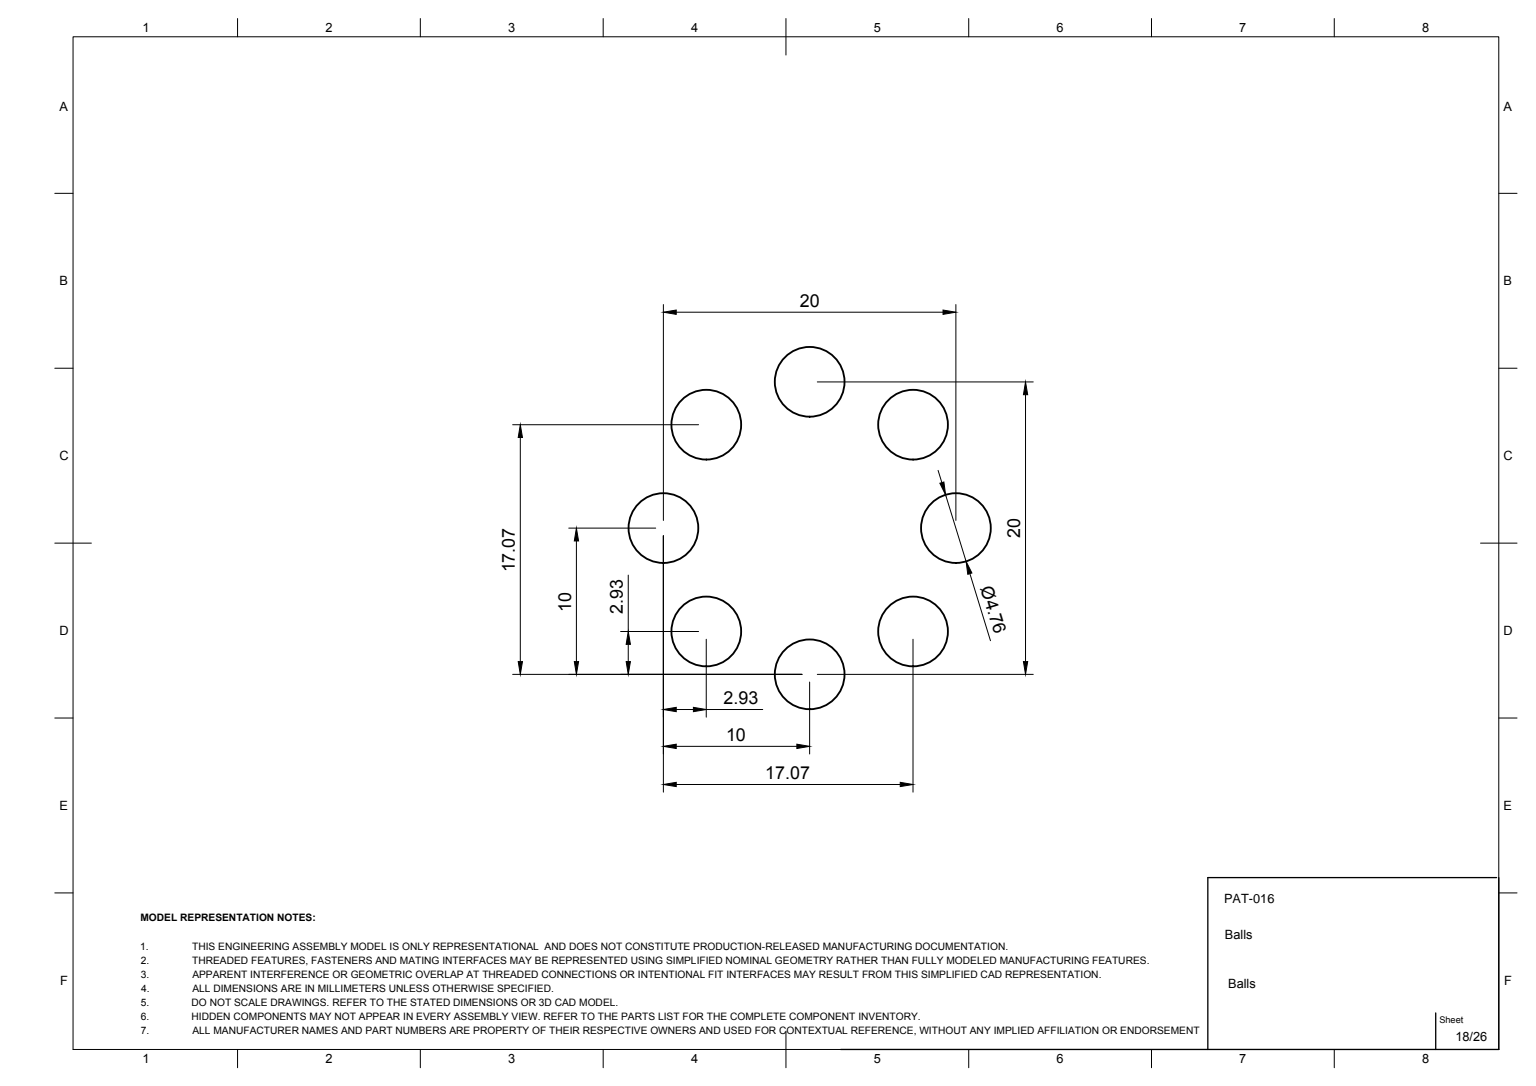
ISO-10303-21;
HEADER;
/* Generated by software containing ST-Developer
 * from STEP Tools, Inc. (www.steptools.com) 
 */

FILE_DESCRIPTION(
/* description */ ('Bracket-mounted idler roller'),
/* implementation_level */ '2;1');

FILE_NAME(
/* name */ 'Balls.step',
/* time_stamp */ '2026-10-28T03:26:42-07:00',
/* author */ (''),
/* organization */ (''),
/* preprocessor_version */ 'ST-DEVELOPER v20.2',
/* originating_system */ 'Autodesk Translation Framework v15.17.0.0',
/* authorisation */ '');

FILE_SCHEMA (('AUTOMOTIVE_DESIGN { 1 0 10303 214 3 1 1 }'));
ENDSEC;

DATA;
#10=MECHANICAL_DESIGN_GEOMETRIC_PRESENTATION_REPRESENTATION('',(#293,#294,#295,#296,#297,#298,#299,#300),#6241);
#205=SPHERICAL_SURFACE('',#3648,0.23815);
#206=SPHERICAL_SURFACE('',#3650,0.23815);
#207=SPHERICAL_SURFACE('',#3652,0.23815);
#208=SPHERICAL_SURFACE('',#3654,0.23815);
#209=SPHERICAL_SURFACE('',#3656,0.23815);
#210=SPHERICAL_SURFACE('',#3658,0.23815);
#211=SPHERICAL_SURFACE('',#3660,0.23815);
#212=SPHERICAL_SURFACE('',#3662,0.23815);
#251=SHAPE_REPRESENTATION_RELATIONSHIP('SRR','None',#6356,#272);
#272=ADVANCED_BREP_SHAPE_REPRESENTATION('',(#321,#322,#323,#324,#325,#326,
#327,#328),#6232);
#293=STYLED_ITEM('',(#6538),#321);
#294=STYLED_ITEM('',(#6538),#322);
#295=STYLED_ITEM('',(#6538),#323);
#296=STYLED_ITEM('',(#6538),#324);
#297=STYLED_ITEM('',(#6538),#325);
#298=STYLED_ITEM('',(#6538),#326);
#299=STYLED_ITEM('',(#6538),#327);
#300=STYLED_ITEM('',(#6538),#328);
#321=MANIFOLD_SOLID_BREP('Body1',#3196);
#322=MANIFOLD_SOLID_BREP('Body2',#3197);
#323=MANIFOLD_SOLID_BREP('Body3',#3198);
#324=MANIFOLD_SOLID_BREP('Body4',#3199);
#325=MANIFOLD_SOLID_BREP('Body5',#3200);
#326=MANIFOLD_SOLID_BREP('Body6',#3201);
#327=MANIFOLD_SOLID_BREP('Body7',#3202);
#328=MANIFOLD_SOLID_BREP('Body8',#3203);
#623=FACE_OUTER_BOUND('',#855,.T.);
#624=FACE_OUTER_BOUND('',#856,.T.);
#625=FACE_OUTER_BOUND('',#857,.T.);
#626=FACE_OUTER_BOUND('',#858,.T.);
#627=FACE_OUTER_BOUND('',#859,.T.);
#628=FACE_OUTER_BOUND('',#860,.T.);
#629=FACE_OUTER_BOUND('',#861,.T.);
#630=FACE_OUTER_BOUND('',#862,.T.);
#855=EDGE_LOOP('',(#2584,#2585));
#856=EDGE_LOOP('',(#2586,#2587));
#857=EDGE_LOOP('',(#2588,#2589));
#858=EDGE_LOOP('',(#2590,#2591));
#859=EDGE_LOOP('',(#2592,#2593));
#860=EDGE_LOOP('',(#2594,#2595));
#861=EDGE_LOOP('',(#2596,#2597));
#862=EDGE_LOOP('',(#2598,#2599));
#1422=CIRCLE('',#3649,0.23815);
#1423=CIRCLE('',#3651,0.23815);
#1424=CIRCLE('',#3653,0.23815);
#1425=CIRCLE('',#3655,0.23815);
#1426=CIRCLE('',#3657,0.23815);
#1427=CIRCLE('',#3659,0.23815);
#1428=CIRCLE('',#3661,0.23815);
#1429=CIRCLE('',#3663,0.23815);
#1661=VERTEX_POINT('',#5421);
#1662=VERTEX_POINT('',#5422);
#1663=VERTEX_POINT('',#5425);
#1664=VERTEX_POINT('',#5426);
#1665=VERTEX_POINT('',#5429);
#1666=VERTEX_POINT('',#5430);
#1667=VERTEX_POINT('',#5433);
#1668=VERTEX_POINT('',#5434);
#1669=VERTEX_POINT('',#5437);
#1670=VERTEX_POINT('',#5438);
#1671=VERTEX_POINT('',#5441);
#1672=VERTEX_POINT('',#5442);
#1673=VERTEX_POINT('',#5445);
#1674=VERTEX_POINT('',#5446);
#1675=VERTEX_POINT('',#5449);
#1676=VERTEX_POINT('',#5450);
#1994=EDGE_CURVE('',#1661,#1662,#1422,.T.);
#1995=EDGE_CURVE('',#1663,#1664,#1423,.T.);
#1996=EDGE_CURVE('',#1665,#1666,#1424,.T.);
#1997=EDGE_CURVE('',#1667,#1668,#1425,.T.);
#1998=EDGE_CURVE('',#1669,#1670,#1426,.T.);
#1999=EDGE_CURVE('',#1671,#1672,#1427,.T.);
#2000=EDGE_CURVE('',#1673,#1674,#1428,.T.);
#2001=EDGE_CURVE('',#1675,#1676,#1429,.T.);
#2584=ORIENTED_EDGE('',*,*,#1994,.T.);
#2585=ORIENTED_EDGE('',*,*,#1994,.F.);
#2586=ORIENTED_EDGE('',*,*,#1995,.T.);
#2587=ORIENTED_EDGE('',*,*,#1995,.F.);
#2588=ORIENTED_EDGE('',*,*,#1996,.T.);
#2589=ORIENTED_EDGE('',*,*,#1996,.F.);
#2590=ORIENTED_EDGE('',*,*,#1997,.T.);
#2591=ORIENTED_EDGE('',*,*,#1997,.F.);
#2592=ORIENTED_EDGE('',*,*,#1998,.T.);
#2593=ORIENTED_EDGE('',*,*,#1998,.F.);
#2594=ORIENTED_EDGE('',*,*,#1999,.T.);
#2595=ORIENTED_EDGE('',*,*,#1999,.F.);
#2596=ORIENTED_EDGE('',*,*,#2000,.T.);
#2597=ORIENTED_EDGE('',*,*,#2000,.F.);
#2598=ORIENTED_EDGE('',*,*,#2001,.T.);
#2599=ORIENTED_EDGE('',*,*,#2001,.F.);
#3098=ADVANCED_FACE('',(#623),#205,.T.);
#3099=ADVANCED_FACE('',(#624),#206,.T.);
#3100=ADVANCED_FACE('',(#625),#207,.T.);
#3101=ADVANCED_FACE('',(#626),#208,.T.);
#3102=ADVANCED_FACE('',(#627),#209,.T.);
#3103=ADVANCED_FACE('',(#628),#210,.T.);
#3104=ADVANCED_FACE('',(#629),#211,.T.);
#3105=ADVANCED_FACE('',(#630),#212,.T.);
#3196=CLOSED_SHELL('',(#3098));
#3197=CLOSED_SHELL('',(#3099));
#3198=CLOSED_SHELL('',(#3100));
#3199=CLOSED_SHELL('',(#3101));
#3200=CLOSED_SHELL('',(#3102));
#3201=CLOSED_SHELL('',(#3103));
#3202=CLOSED_SHELL('',(#3104));
#3203=CLOSED_SHELL('',(#3105));
#3647=AXIS2_PLACEMENT_3D('',#5419,#4420,#4421);
#3648=AXIS2_PLACEMENT_3D('',#5420,#4422,#4423);
#3649=AXIS2_PLACEMENT_3D('',#5423,#4424,#4425);
#3650=AXIS2_PLACEMENT_3D('',#5424,#4426,#4427);
#3651=AXIS2_PLACEMENT_3D('',#5427,#4428,#4429);
#3652=AXIS2_PLACEMENT_3D('',#5428,#4430,#4431);
#3653=AXIS2_PLACEMENT_3D('',#5431,#4432,#4433);
#3654=AXIS2_PLACEMENT_3D('',#5432,#4434,#4435);
#3655=AXIS2_PLACEMENT_3D('',#5435,#4436,#4437);
#3656=AXIS2_PLACEMENT_3D('',#5436,#4438,#4439);
#3657=AXIS2_PLACEMENT_3D('',#5439,#4440,#4441);
#3658=AXIS2_PLACEMENT_3D('',#5440,#4442,#4443);
#3659=AXIS2_PLACEMENT_3D('',#5443,#4444,#4445);
#3660=AXIS2_PLACEMENT_3D('',#5444,#4446,#4447);
#3661=AXIS2_PLACEMENT_3D('',#5447,#4448,#4449);
#3662=AXIS2_PLACEMENT_3D('',#5448,#4450,#4451);
#3663=AXIS2_PLACEMENT_3D('',#5451,#4452,#4453);
#4420=DIRECTION('axis',(0.,0.,1.));
#4421=DIRECTION('refdir',(1.,0.,0.));
#4422=DIRECTION('center_axis',(0.,0.,1.));
#4423=DIRECTION('ref_axis',(1.,0.,0.));
#4424=DIRECTION('center_axis',(1.22464679914735E-16,-1.,0.));
#4425=DIRECTION('ref_axis',(-1.,-1.22464679914735E-16,0.));
#4426=DIRECTION('center_axis',(0.707106781186548,0.,0.707106781186548));
#4427=DIRECTION('ref_axis',(0.707106781186548,0.,-0.707106781186548));
#4428=DIRECTION('center_axis',(8.65956056235494E-17,-1.,-8.65956056235493E-17));
#4429=DIRECTION('ref_axis',(-0.707106781186547,-1.22464679914735E-16,0.707106781186547));
#4430=DIRECTION('center_axis',(1.,0.,0.));
#4431=DIRECTION('ref_axis',(6.12323399573676E-17,0.,-1.));
#4432=DIRECTION('center_axis',(7.49879891330929E-33,-1.,-1.22464679914735E-16));
#4433=DIRECTION('ref_axis',(-6.12323399573676E-17,-1.22464679914735E-16,
1.));
#4434=DIRECTION('center_axis',(0.707106781186548,0.,-0.707106781186548));
#4435=DIRECTION('ref_axis',(-0.707106781186548,0.,-0.707106781186548));
#4436=DIRECTION('center_axis',(-8.65956056235493E-17,-1.,-8.65956056235494E-17));
#4437=DIRECTION('ref_axis',(0.707106781186547,-1.22464679914735E-16,0.707106781186547));
#4438=DIRECTION('center_axis',(0.,0.,-1.));
#4439=DIRECTION('ref_axis',(-1.,0.,-1.22464679914735E-16));
#4440=DIRECTION('center_axis',(-1.22464679914735E-16,-1.,-1.49975978266186E-32));
#4441=DIRECTION('ref_axis',(1.,-1.22464679914735E-16,1.22464679914735E-16));
#4442=DIRECTION('center_axis',(-0.707106781186547,0.,-0.707106781186548));
#4443=DIRECTION('ref_axis',(-0.707106781186548,0.,0.707106781186547));
#4444=DIRECTION('center_axis',(-8.65956056235493E-17,-1.,8.65956056235493E-17));
#4445=DIRECTION('ref_axis',(0.707106781186548,-1.22464679914735E-16,-0.707106781186547));
#4446=DIRECTION('center_axis',(-1.,0.,0.));
#4447=DIRECTION('ref_axis',(-1.83697019872103E-16,0.,1.));
#4448=DIRECTION('center_axis',(-2.24963967399279E-32,-1.,1.22464679914735E-16));
#4449=DIRECTION('ref_axis',(1.83697019872103E-16,-1.22464679914735E-16,
-1.));
#4450=DIRECTION('center_axis',(-0.707106781186548,0.,0.707106781186548));
#4451=DIRECTION('ref_axis',(0.707106781186547,0.,0.707106781186548));
#4452=DIRECTION('center_axis',(8.65956056235493E-17,-1.,8.65956056235493E-17));
#4453=DIRECTION('ref_axis',(-0.707106781186547,-1.22464679914735E-16,-0.707106781186548));
#5419=CARTESIAN_POINT('',(0.,0.,0.));
#5420=CARTESIAN_POINT('Origin',(1.,0.,0.));
#5421=CARTESIAN_POINT('',(1.,-1.78583896120461E-33,0.23815));
#5422=CARTESIAN_POINT('',(1.,-1.78583896120461E-33,-0.23815));
#5423=CARTESIAN_POINT('Origin',(1.,0.,0.));
#5424=CARTESIAN_POINT('Origin',(0.707106781186548,0.,-0.707106781186547));
#5425=CARTESIAN_POINT('',(0.875504261126124,-1.78583896120461E-33,-0.538709301246971));
#5426=CARTESIAN_POINT('',(0.538709301246971,-1.78583896120461E-33,-0.875504261126124));
#5427=CARTESIAN_POINT('Origin',(0.707106781186548,0.,-0.707106781186547));
#5428=CARTESIAN_POINT('Origin',(6.12323399573677E-17,0.,-1.));
#5429=CARTESIAN_POINT('',(0.23815,-1.78583896120461E-33,-1.));
#5430=CARTESIAN_POINT('',(-0.23815,-1.78583896120461E-33,-1.));
#5431=CARTESIAN_POINT('Origin',(6.12323399573677E-17,0.,-1.));
#5432=CARTESIAN_POINT('Origin',(-0.707106781186547,0.,-0.707106781186548));
#5433=CARTESIAN_POINT('',(-0.538709301246971,-1.78583896120461E-33,-0.875504261126124));
#5434=CARTESIAN_POINT('',(-0.875504261126124,-1.78583896120461E-33,-0.538709301246971));
#5435=CARTESIAN_POINT('Origin',(-0.707106781186547,0.,-0.707106781186548));
#5436=CARTESIAN_POINT('Origin',(-1.,0.,-1.22464679914735E-16));
#5437=CARTESIAN_POINT('',(-1.,-1.78583896120461E-33,-0.23815));
#5438=CARTESIAN_POINT('',(-1.,-1.78583896120461E-33,0.23815));
#5439=CARTESIAN_POINT('Origin',(-1.,0.,-1.22464679914735E-16));
#5440=CARTESIAN_POINT('Origin',(-0.707106781186548,0.,0.707106781186547));
#5441=CARTESIAN_POINT('',(-0.875504261126124,-7.94881478324376E-33,0.538709301246971));
#5442=CARTESIAN_POINT('',(-0.538709301246971,4.37713686083455E-33,0.875504261126124));
#5443=CARTESIAN_POINT('Origin',(-0.707106781186548,0.,0.707106781186547));
#5444=CARTESIAN_POINT('Origin',(-1.83697019872103E-16,0.,1.));
#5445=CARTESIAN_POINT('',(-0.23815,-1.78583896120461E-33,1.));
#5446=CARTESIAN_POINT('',(0.23815,-1.78583896120461E-33,1.));
#5447=CARTESIAN_POINT('Origin',(-1.83697019872103E-16,0.,1.));
#5448=CARTESIAN_POINT('Origin',(0.707106781186547,0.,0.707106781186548));
#5449=CARTESIAN_POINT('',(0.538709301246971,-4.86732687222419E-33,0.875504261126124));
#5450=CARTESIAN_POINT('',(0.875504261126124,1.29564894981497E-33,0.538709301246971));
#5451=CARTESIAN_POINT('Origin',(0.707106781186547,0.,0.707106781186548));
#6206=UNCERTAINTY_MEASURE_WITH_UNIT(LENGTH_MEASURE(0.001),#6242,
'DISTANCE_ACCURACY_VALUE',
'Maximum model space distance between geometric entities at asserted c
onnectivities');
#6215=UNCERTAINTY_MEASURE_WITH_UNIT(LENGTH_MEASURE(0.001),#6242,
'DISTANCE_ACCURACY_VALUE',
'Maximum model space distance between geometric entities at asserted c
onnectivities');
#6232=(
GEOMETRIC_REPRESENTATION_CONTEXT(3)
GLOBAL_UNCERTAINTY_ASSIGNED_CONTEXT((#6206))
GLOBAL_UNIT_ASSIGNED_CONTEXT((#6242,#6244,#6245))
REPRESENTATION_CONTEXT('','3D')
);
#6241=(
GEOMETRIC_REPRESENTATION_CONTEXT(3)
GLOBAL_UNCERTAINTY_ASSIGNED_CONTEXT((#6215))
GLOBAL_UNIT_ASSIGNED_CONTEXT((#6242,#6244,#6245))
REPRESENTATION_CONTEXT('','3D')
);
#6242=(
LENGTH_UNIT()
NAMED_UNIT(*)
SI_UNIT(.CENTI.,.METRE.)
);
#6244=(
NAMED_UNIT(*)
PLANE_ANGLE_UNIT()
SI_UNIT($,.RADIAN.)
);
#6245=(
NAMED_UNIT(*)
SI_UNIT($,.STERADIAN.)
SOLID_ANGLE_UNIT()
);
#6262=SHAPE_DEFINITION_REPRESENTATION(#6287,#6356);
#6287=PRODUCT_DEFINITION_SHAPE('',$,#6382);
#6356=SHAPE_REPRESENTATION('',(#3647),#6232);
#6365=PRODUCT_DEFINITION_CONTEXT('part definition',#6442,'design');
#6382=PRODUCT_DEFINITION('Balls','Balls',#6407,#6365);
#6407=PRODUCT_DEFINITION_FORMATION('',$,#6460);
#6442=APPLICATION_CONTEXT(
'Core Data for Automotive Mechanical Design Process');
#6443=PRODUCT_CONTEXT('part definition',#6442,'mechanical');
#6460=PRODUCT('Balls','Balls','Balls',(#6443));
#6532=COLOUR_RGB('Grey',0.48,0.52,0.57);
#6533=FILL_AREA_STYLE_COLOUR('',#6532);
#6534=FILL_AREA_STYLE('',(#6533));
#6535=SURFACE_STYLE_FILL_AREA(#6534);
#6536=SURFACE_SIDE_STYLE('',(#6535));
#6537=SURFACE_STYLE_USAGE(.BOTH.,#6536);
#6538=PRESENTATION_STYLE_ASSIGNMENT((#6537));
ENDSEC;
END-ISO-10303-21;
